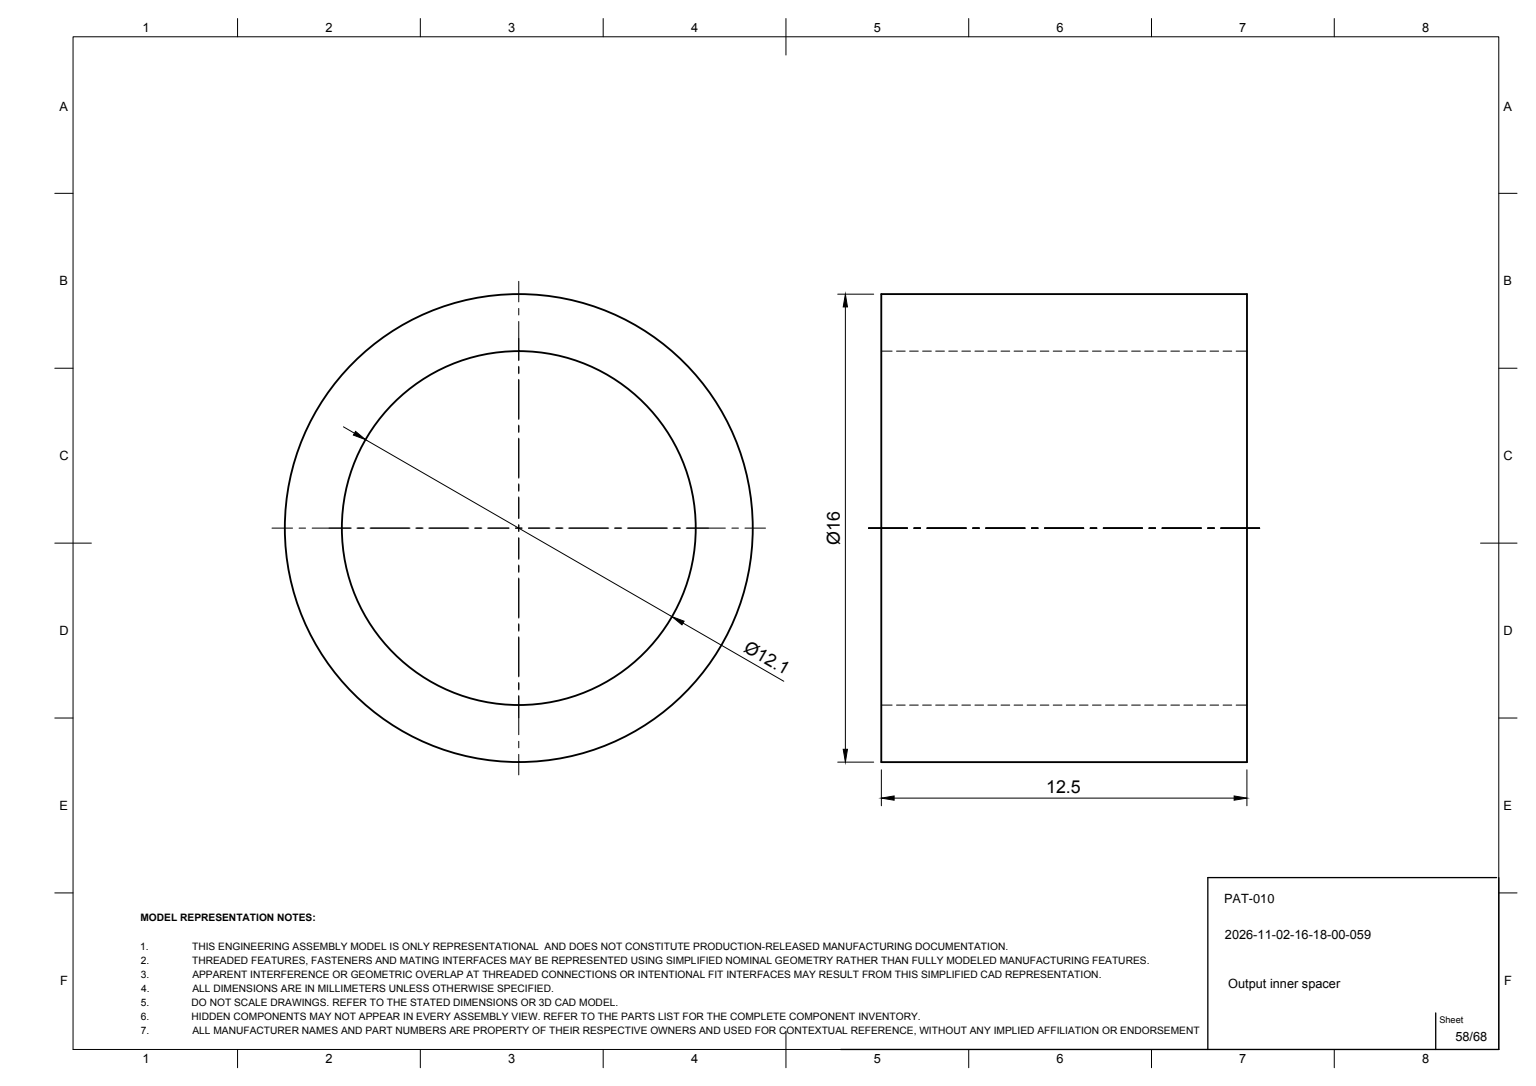
ISO-10303-21;
HEADER;
/* Generated by software containing ST-Developer
 * from STEP Tools, Inc. (www.steptools.com) 
 */

FILE_DESCRIPTION(
/* description */ ('Belt conveyor head drive unit'),
/* implementation_level */ '2;1');

FILE_NAME(
/* name */ 'Output inner spacer.step',
/* time_stamp */ '2026-10-28T03:26:19-07:00',
/* author */ (''),
/* organization */ (''),
/* preprocessor_version */ 'ST-DEVELOPER v20.2',
/* originating_system */ 'Autodesk Translation Framework v15.17.0.0',
/* authorisation */ '');

FILE_SCHEMA (('AUTOMOTIVE_DESIGN { 1 0 10303 214 3 1 1 }'));
ENDSEC;

DATA;
#10=MECHANICAL_DESIGN_GEOMETRIC_PRESENTATION_REPRESENTATION('',(#917),#27069);
#763=SHAPE_REPRESENTATION_RELATIONSHIP('SRR','None',#27412,#832);
#832=ADVANCED_BREP_SHAPE_REPRESENTATION('',(#998),#27054);
#917=STYLED_ITEM('',(#27790),#998);
#998=MANIFOLD_SOLID_BREP('Body1',#13786);
#1236=FACE_BOUND('',#3280,.T.);
#1237=FACE_BOUND('',#3282,.T.);
#1576=PLANE('',#15897);
#1577=PLANE('',#15898);
#2253=FACE_OUTER_BOUND('',#3277,.T.);
#2254=FACE_OUTER_BOUND('',#3278,.T.);
#2255=FACE_OUTER_BOUND('',#3279,.T.);
#2256=FACE_OUTER_BOUND('',#3281,.T.);
#3277=EDGE_LOOP('',(#11646,#11647,#11648,#11649));
#3278=EDGE_LOOP('',(#11650,#11651,#11652,#11653));
#3279=EDGE_LOOP('',(#11654));
#3280=EDGE_LOOP('',(#11655));
#3281=EDGE_LOOP('',(#11656));
#3282=EDGE_LOOP('',(#11657));
#4121=LINE('',#25354,#4913);
#4122=LINE('',#25360,#4914);
#4913=VECTOR('',#19719,0.605);
#4914=VECTOR('',#19726,0.8);
#5717=CIRCLE('',#15892,0.605);
#5718=CIRCLE('',#15893,0.605);
#5719=CIRCLE('',#15895,0.8);
#5720=CIRCLE('',#15896,0.8);
#6873=VERTEX_POINT('',#25351);
#6874=VERTEX_POINT('',#25353);
#6875=VERTEX_POINT('',#25357);
#6876=VERTEX_POINT('',#25359);
#8515=EDGE_CURVE('',#6873,#6873,#5717,.T.);
#8516=EDGE_CURVE('',#6873,#6874,#4121,.T.);
#8517=EDGE_CURVE('',#6874,#6874,#5718,.T.);
#8518=EDGE_CURVE('',#6875,#6875,#5719,.T.);
#8519=EDGE_CURVE('',#6875,#6876,#4122,.T.);
#8520=EDGE_CURVE('',#6876,#6876,#5720,.T.);
#11646=ORIENTED_EDGE('',*,*,#8515,.F.);
#11647=ORIENTED_EDGE('',*,*,#8516,.T.);
#11648=ORIENTED_EDGE('',*,*,#8517,.T.);
#11649=ORIENTED_EDGE('',*,*,#8516,.F.);
#11650=ORIENTED_EDGE('',*,*,#8518,.F.);
#11651=ORIENTED_EDGE('',*,*,#8519,.T.);
#11652=ORIENTED_EDGE('',*,*,#8520,.T.);
#11653=ORIENTED_EDGE('',*,*,#8519,.F.);
#11654=ORIENTED_EDGE('',*,*,#8518,.T.);
#11655=ORIENTED_EDGE('',*,*,#8515,.T.);
#11656=ORIENTED_EDGE('',*,*,#8520,.F.);
#11657=ORIENTED_EDGE('',*,*,#8517,.F.);
#12795=CYLINDRICAL_SURFACE('',#15891,0.605);
#12796=CYLINDRICAL_SURFACE('',#15894,0.8);
#13532=ADVANCED_FACE('',(#2253),#12795,.F.);
#13533=ADVANCED_FACE('',(#2254),#12796,.T.);
#13534=ADVANCED_FACE('',(#2255,#1236),#1576,.T.);
#13535=ADVANCED_FACE('',(#2256,#1237),#1577,.F.);
#13786=CLOSED_SHELL('',(#13532,#13533,#13534,#13535));
#15890=AXIS2_PLACEMENT_3D('',#25349,#19713,#19714);
#15891=AXIS2_PLACEMENT_3D('',#25350,#19715,#19716);
#15892=AXIS2_PLACEMENT_3D('',#25352,#19717,#19718);
#15893=AXIS2_PLACEMENT_3D('',#25355,#19720,#19721);
#15894=AXIS2_PLACEMENT_3D('',#25356,#19722,#19723);
#15895=AXIS2_PLACEMENT_3D('',#25358,#19724,#19725);
#15896=AXIS2_PLACEMENT_3D('',#25361,#19727,#19728);
#15897=AXIS2_PLACEMENT_3D('',#25362,#19729,#19730);
#15898=AXIS2_PLACEMENT_3D('',#25363,#19731,#19732);
#19713=DIRECTION('axis',(0.,0.,1.));
#19714=DIRECTION('refdir',(1.,0.,0.));
#19715=DIRECTION('center_axis',(0.,1.,0.));
#19716=DIRECTION('ref_axis',(1.,0.,0.));
#19717=DIRECTION('center_axis',(0.,-1.,0.));
#19718=DIRECTION('ref_axis',(1.,0.,0.));
#19719=DIRECTION('',(0.,-1.,0.));
#19720=DIRECTION('center_axis',(0.,-1.,0.));
#19721=DIRECTION('ref_axis',(1.,0.,0.));
#19722=DIRECTION('center_axis',(0.,1.,0.));
#19723=DIRECTION('ref_axis',(1.,0.,0.));
#19724=DIRECTION('center_axis',(0.,1.,0.));
#19725=DIRECTION('ref_axis',(1.,0.,0.));
#19726=DIRECTION('',(0.,-1.,0.));
#19727=DIRECTION('center_axis',(0.,1.,0.));
#19728=DIRECTION('ref_axis',(1.,0.,0.));
#19729=DIRECTION('center_axis',(0.,1.,0.));
#19730=DIRECTION('ref_axis',(1.,0.,0.));
#19731=DIRECTION('center_axis',(0.,1.,0.));
#19732=DIRECTION('ref_axis',(1.,0.,0.));
#25349=CARTESIAN_POINT('',(0.,0.,0.));
#25350=CARTESIAN_POINT('Origin',(6.97091003018116,-2.65,7.));
#25351=CARTESIAN_POINT('',(6.36591003018116,-1.4,7.));
#25352=CARTESIAN_POINT('Origin',(6.97091003018116,-1.4,7.));
#25353=CARTESIAN_POINT('',(6.36591003018116,-2.65,7.));
#25354=CARTESIAN_POINT('',(6.36591003018116,-2.65,7.));
#25355=CARTESIAN_POINT('Origin',(6.97091003018116,-2.65,7.));
#25356=CARTESIAN_POINT('Origin',(6.97091003018116,-2.65,7.));
#25357=CARTESIAN_POINT('',(6.17091003018116,-1.4,7.));
#25358=CARTESIAN_POINT('Origin',(6.97091003018116,-1.4,7.));
#25359=CARTESIAN_POINT('',(6.17091003018116,-2.65,7.));
#25360=CARTESIAN_POINT('',(6.17091003018116,-2.65,7.));
#25361=CARTESIAN_POINT('Origin',(6.97091003018116,-2.65,7.));
#25362=CARTESIAN_POINT('Origin',(6.97091003018116,-1.4,7.));
#25363=CARTESIAN_POINT('Origin',(6.97091003018116,-2.65,7.));
#26977=UNCERTAINTY_MEASURE_WITH_UNIT(LENGTH_MEASURE(0.001),#27070,
'DISTANCE_ACCURACY_VALUE',
'Maximum model space distance between geometric entities at asserted c
onnectivities');
#26992=UNCERTAINTY_MEASURE_WITH_UNIT(LENGTH_MEASURE(0.001),#27070,
'DISTANCE_ACCURACY_VALUE',
'Maximum model space distance between geometric entities at asserted c
onnectivities');
#27054=(
GEOMETRIC_REPRESENTATION_CONTEXT(3)
GLOBAL_UNCERTAINTY_ASSIGNED_CONTEXT((#26977))
GLOBAL_UNIT_ASSIGNED_CONTEXT((#27070,#27072,#27073))
REPRESENTATION_CONTEXT('','3D')
);
#27069=(
GEOMETRIC_REPRESENTATION_CONTEXT(3)
GLOBAL_UNCERTAINTY_ASSIGNED_CONTEXT((#26992))
GLOBAL_UNIT_ASSIGNED_CONTEXT((#27070,#27072,#27073))
REPRESENTATION_CONTEXT('','3D')
);
#27070=(
LENGTH_UNIT()
NAMED_UNIT(*)
SI_UNIT(.CENTI.,.METRE.)
);
#27072=(
NAMED_UNIT(*)
PLANE_ANGLE_UNIT()
SI_UNIT($,.RADIAN.)
);
#27073=(
NAMED_UNIT(*)
SI_UNIT($,.STERADIAN.)
SOLID_ANGLE_UNIT()
);
#27135=SHAPE_DEFINITION_REPRESENTATION(#27223,#27412);
#27223=PRODUCT_DEFINITION_SHAPE('',$,#27489);
#27412=SHAPE_REPRESENTATION('',(#15890),#27054);
#27427=PRODUCT_DEFINITION_CONTEXT('part definition',#27657,'design');
#27489=PRODUCT_DEFINITION('Output inner spacer','Output inner spacer',#27565,
#27427);
#27565=PRODUCT_DEFINITION_FORMATION('',$,#27720);
#27657=APPLICATION_CONTEXT(
'Core Data for Automotive Mechanical Design Process');
#27658=PRODUCT_CONTEXT('part definition',#27657,'mechanical');
#27720=PRODUCT('Output inner spacer','Output inner spacer',
'Output inner spacer',(#27658));
#27784=COLOUR_RGB('Sky Blue',0.24,0.69,0.87);
#27785=FILL_AREA_STYLE_COLOUR('',#27784);
#27786=FILL_AREA_STYLE('',(#27785));
#27787=SURFACE_STYLE_FILL_AREA(#27786);
#27788=SURFACE_SIDE_STYLE('',(#27787));
#27789=SURFACE_STYLE_USAGE(.BOTH.,#27788);
#27790=PRESENTATION_STYLE_ASSIGNMENT((#27789));
ENDSEC;
END-ISO-10303-21;
